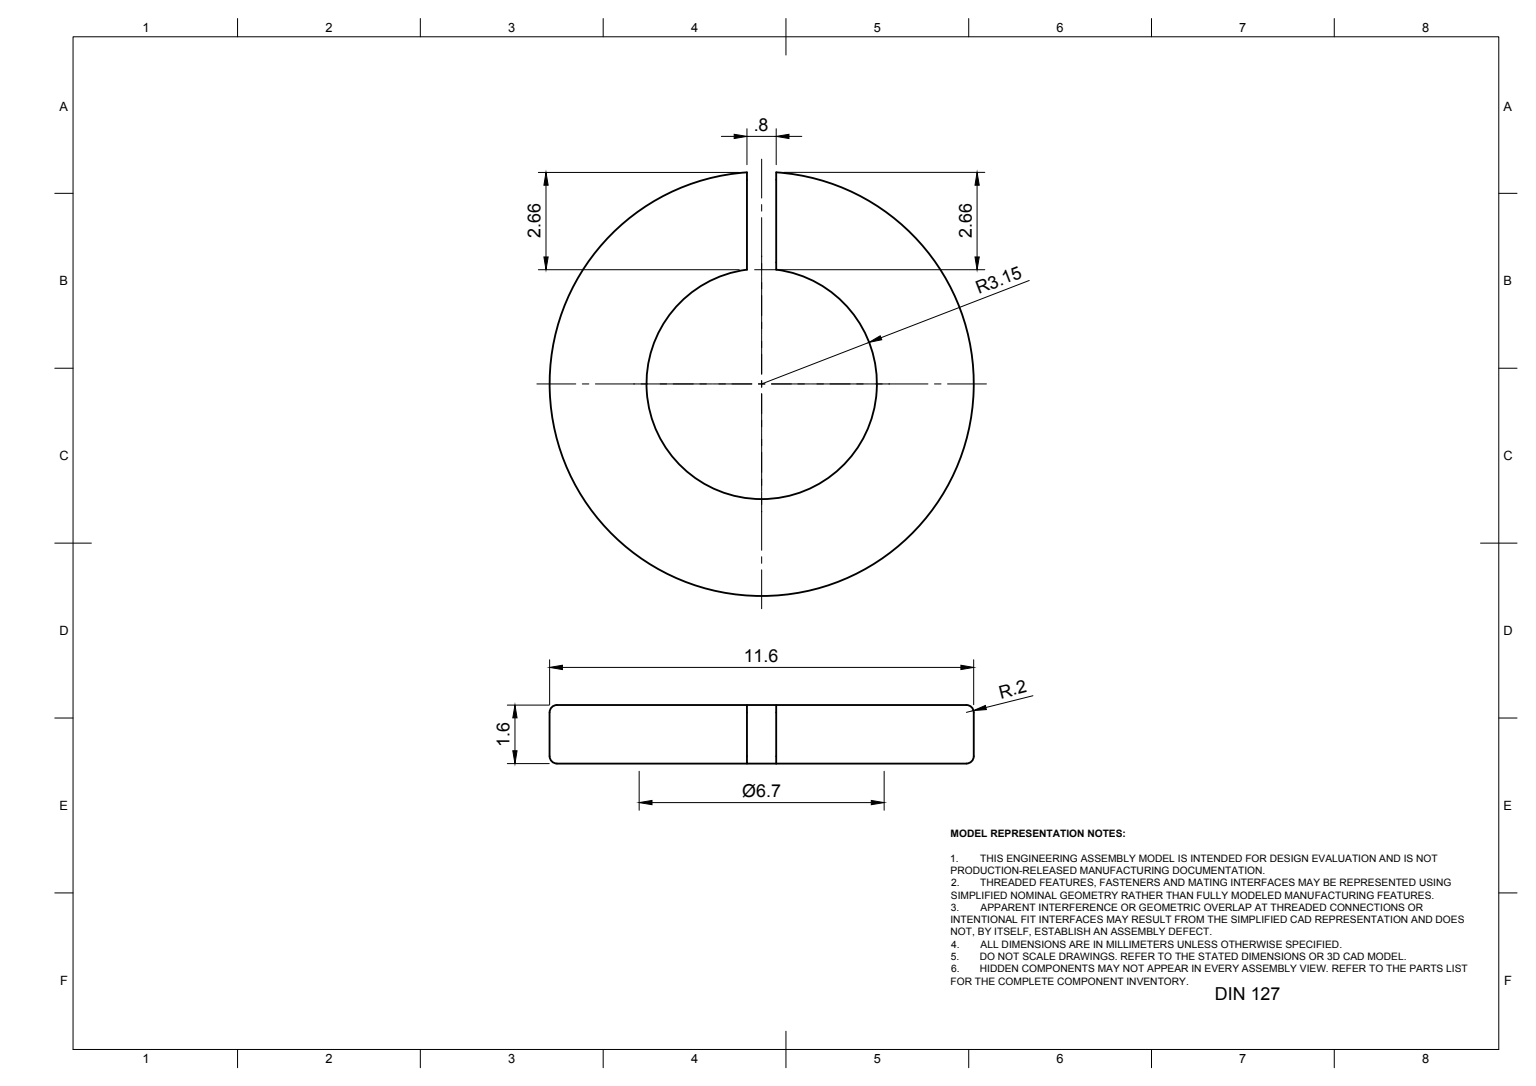
ISO-10303-21;
HEADER;
/* Generated by software containing ST-Developer
 * from STEP Tools, Inc. (www.steptools.com) 
 */

FILE_DESCRIPTION(
/* description */ ('STEP AP214'),
/* implementation_level */ '2;1');

FILE_NAME(
/* name */ 'DIN 127.step',
/* time_stamp */ '2026-10-07T12:18:07-07:00',
/* author */ (''),
/* organization */ (''),
/* preprocessor_version */ 'ST-DEVELOPER v20.2',
/* originating_system */ 'Autodesk Translation Framework v15.15.0.0',
/* authorisation */ '');

FILE_SCHEMA (('AUTOMOTIVE_DESIGN { 1 0 10303 214 3 1 1 }'));
ENDSEC;

DATA;
#10=MECHANICAL_DESIGN_GEOMETRIC_PRESENTATION_REPRESENTATION('',(#132),#62974);
#108=SHAPE_REPRESENTATION_RELATIONSHIP('SRR','None',#63031,#120);
#120=ADVANCED_BREP_SHAPE_REPRESENTATION('',(#144),#62972);
#132=STYLED_ITEM('',(#63090),#144);
#144=MANIFOLD_SOLID_BREP('Body1',#15202);
#716=PLANE('',#16878);
#717=PLANE('',#16879);
#718=PLANE('',#16882);
#719=PLANE('',#16883);
#1024=B_SPLINE_CURVE_WITH_KNOTS('',3,(#62662,#62663,#62664,#62665,#62666,
#62667,#62668,#62669,#62670,#62671),.UNSPECIFIED.,.F.,.F.,(4,2,2,2,4),(-0.0891808869303931,
-0.0817048501723883,-0.0742536419552704,-0.0668368032479844,-0.0594502997646748),
 .UNSPECIFIED.);
#1025=B_SPLINE_CURVE_WITH_KNOTS('',3,(#62674,#62675,#62676,#62677,#62678,
#62679,#62680,#62681,#62682,#62683),.UNSPECIFIED.,.F.,.F.,(4,2,2,2,4),(0.0594551317141721,
0.0668412192577732,0.0742583320696144,0.081710598423227,0.0891882604952256),
 .UNSPECIFIED.);
#1026=B_SPLINE_CURVE_WITH_KNOTS('',3,(#62689,#62690,#62691,#62692,#62693,
#62694,#62695,#62696,#62697,#62698),.UNSPECIFIED.,.F.,.F.,(4,2,2,2,4),(0.,
0.0073991168916538,0.0148071582868911,0.022226415171961,0.0296556575450588),
 .UNSPECIFIED.);
#1027=B_SPLINE_CURVE_WITH_KNOTS('',3,(#62701,#62702,#62703,#62704,#62705,
#62706,#62707,#62708,#62709,#62710),.UNSPECIFIED.,.F.,.F.,(4,2,2,2,4),(0.0889741245006404,
0.0964039199286515,0.103823503599454,0.111231617988348,0.118630606154988),
 .UNSPECIFIED.);
#1028=B_SPLINE_CURVE_WITH_KNOTS('',3,(#62716,#62717,#62718,#62719,#62720,
#62721,#62722,#62723,#62724,#62725),.UNSPECIFIED.,.F.,.F.,(4,2,2,2,4),(0.0889715481092505,
0.0964007904823484,0.103820047367418,0.111228088762656,0.118627205654309),
 .UNSPECIFIED.);
#1029=B_SPLINE_CURVE_WITH_KNOTS('',3,(#62728,#62729,#62730,#62731,#62732,
#62733,#62734,#62735,#62736,#62737),.UNSPECIFIED.,.F.,.F.,(4,2,2,2,4),(0.,
0.00739898816663991,0.014807102555534,0.0222266862263364,0.0296564816543475),
 .UNSPECIFIED.);
#1030=B_SPLINE_CURVE_WITH_KNOTS('',3,(#62743,#62744,#62745,#62746,#62747,
#62748,#62749,#62750,#62751,#62752),.UNSPECIFIED.,.F.,.F.,(4,2,2,2,4),(0.0594502997646748,
0.0668368032479844,0.0742536419552704,0.0817048501723883,0.0891808869303931),
 .UNSPECIFIED.);
#1031=B_SPLINE_CURVE_WITH_KNOTS('',3,(#62755,#62756,#62757,#62758,#62759,
#62760,#62761,#62762,#62763,#62764),.UNSPECIFIED.,.F.,.F.,(4,2,2,2,4),(0.0297220029331187,
0.0371996650051172,0.0446519313587299,0.0520690441705711,0.0594551317141721),
 .UNSPECIFIED.);
#2207=LINE('',#62766,#3400);
#2208=LINE('',#62767,#3401);
#2209=LINE('',#62769,#3402);
#2210=LINE('',#62770,#3403);
#2211=LINE('',#62772,#3404);
#2212=LINE('',#62773,#3405);
#2213=LINE('',#62775,#3406);
#2214=LINE('',#62776,#3407);
#3400=VECTOR('',#21190,1000.);
#3401=VECTOR('',#21191,1000.);
#3402=VECTOR('',#21194,1000.);
#3403=VECTOR('',#21195,1000.);
#3404=VECTOR('',#21198,1000.);
#3405=VECTOR('',#21199,1000.);
#3406=VECTOR('',#21202,1000.);
#3407=VECTOR('',#21203,1000.);
#3686=CYLINDRICAL_SURFACE('',#16880,3.15);
#3687=CYLINDRICAL_SURFACE('',#16881,5.8);
#4518=FACE_OUTER_BOUND('',#5468,.T.);
#4519=FACE_OUTER_BOUND('',#5469,.T.);
#4520=FACE_OUTER_BOUND('',#5470,.T.);
#4521=FACE_OUTER_BOUND('',#5471,.T.);
#4522=FACE_OUTER_BOUND('',#5472,.T.);
#4523=FACE_OUTER_BOUND('',#5473,.T.);
#4524=FACE_OUTER_BOUND('',#5474,.T.);
#4525=FACE_OUTER_BOUND('',#5475,.T.);
#4526=FACE_OUTER_BOUND('',#5476,.T.);
#4527=FACE_OUTER_BOUND('',#5477,.T.);
#5468=EDGE_LOOP('',(#14069,#14070,#14071,#14072));
#5469=EDGE_LOOP('',(#14073,#14074,#14075,#14076));
#5470=EDGE_LOOP('',(#14077,#14078,#14079,#14080));
#5471=EDGE_LOOP('',(#14081,#14082,#14083,#14084));
#5472=EDGE_LOOP('',(#14085,#14086,#14087,#14088));
#5473=EDGE_LOOP('',(#14089,#14090,#14091,#14092));
#5474=EDGE_LOOP('',(#14093,#14094,#14095,#14096));
#5475=EDGE_LOOP('',(#14097,#14098,#14099,#14100));
#5476=EDGE_LOOP('',(#14101,#14102,#14103,#14104,#14105,#14106,#14107,#14108));
#5477=EDGE_LOOP('',(#14109,#14110,#14111,#14112,#14113,#14114,#14115,#14116));
#6186=CIRCLE('',#16867,3.15);
#6187=CIRCLE('',#16868,3.35);
#6188=CIRCLE('',#16870,5.6);
#6189=CIRCLE('',#16871,5.8);
#6190=CIRCLE('',#16873,5.8);
#6191=CIRCLE('',#16874,5.6);
#6192=CIRCLE('',#16876,3.35);
#6193=CIRCLE('',#16877,3.15);
#7564=VERTEX_POINT('',#62658);
#7565=VERTEX_POINT('',#62659);
#7566=VERTEX_POINT('',#62661);
#7567=VERTEX_POINT('',#62672);
#7568=VERTEX_POINT('',#62685);
#7569=VERTEX_POINT('',#62686);
#7570=VERTEX_POINT('',#62688);
#7571=VERTEX_POINT('',#62699);
#7572=VERTEX_POINT('',#62712);
#7573=VERTEX_POINT('',#62713);
#7574=VERTEX_POINT('',#62715);
#7575=VERTEX_POINT('',#62726);
#7576=VERTEX_POINT('',#62739);
#7577=VERTEX_POINT('',#62740);
#7578=VERTEX_POINT('',#62742);
#7579=VERTEX_POINT('',#62753);
#9741=EDGE_CURVE('',#7564,#7565,#6186,.T.);
#9742=EDGE_CURVE('',#7566,#7564,#1024,.T.);
#9743=EDGE_CURVE('',#7567,#7566,#6187,.T.);
#9744=EDGE_CURVE('',#7565,#7567,#1025,.T.);
#9745=EDGE_CURVE('',#7568,#7569,#6188,.T.);
#9746=EDGE_CURVE('',#7570,#7568,#1026,.T.);
#9747=EDGE_CURVE('',#7571,#7570,#6189,.T.);
#9748=EDGE_CURVE('',#7569,#7571,#1027,.T.);
#9749=EDGE_CURVE('',#7572,#7573,#6190,.T.);
#9750=EDGE_CURVE('',#7574,#7572,#1028,.T.);
#9751=EDGE_CURVE('',#7575,#7574,#6191,.T.);
#9752=EDGE_CURVE('',#7573,#7575,#1029,.T.);
#9753=EDGE_CURVE('',#7576,#7577,#6192,.T.);
#9754=EDGE_CURVE('',#7578,#7576,#1030,.T.);
#9755=EDGE_CURVE('',#7579,#7578,#6193,.T.);
#9756=EDGE_CURVE('',#7577,#7579,#1031,.T.);
#9757=EDGE_CURVE('',#7567,#7569,#2207,.T.);
#9758=EDGE_CURVE('',#7568,#7566,#2208,.T.);
#9759=EDGE_CURVE('',#7577,#7575,#2209,.T.);
#9760=EDGE_CURVE('',#7574,#7576,#2210,.T.);
#9761=EDGE_CURVE('',#7578,#7564,#2211,.T.);
#9762=EDGE_CURVE('',#7579,#7565,#2212,.T.);
#9763=EDGE_CURVE('',#7572,#7570,#2213,.T.);
#9764=EDGE_CURVE('',#7573,#7571,#2214,.T.);
#14069=ORIENTED_EDGE('',*,*,#9741,.F.);
#14070=ORIENTED_EDGE('',*,*,#9742,.F.);
#14071=ORIENTED_EDGE('',*,*,#9743,.F.);
#14072=ORIENTED_EDGE('',*,*,#9744,.F.);
#14073=ORIENTED_EDGE('',*,*,#9745,.F.);
#14074=ORIENTED_EDGE('',*,*,#9746,.F.);
#14075=ORIENTED_EDGE('',*,*,#9747,.F.);
#14076=ORIENTED_EDGE('',*,*,#9748,.F.);
#14077=ORIENTED_EDGE('',*,*,#9749,.F.);
#14078=ORIENTED_EDGE('',*,*,#9750,.F.);
#14079=ORIENTED_EDGE('',*,*,#9751,.F.);
#14080=ORIENTED_EDGE('',*,*,#9752,.F.);
#14081=ORIENTED_EDGE('',*,*,#9753,.F.);
#14082=ORIENTED_EDGE('',*,*,#9754,.F.);
#14083=ORIENTED_EDGE('',*,*,#9755,.F.);
#14084=ORIENTED_EDGE('',*,*,#9756,.F.);
#14085=ORIENTED_EDGE('',*,*,#9757,.F.);
#14086=ORIENTED_EDGE('',*,*,#9743,.T.);
#14087=ORIENTED_EDGE('',*,*,#9758,.F.);
#14088=ORIENTED_EDGE('',*,*,#9745,.T.);
#14089=ORIENTED_EDGE('',*,*,#9759,.T.);
#14090=ORIENTED_EDGE('',*,*,#9751,.T.);
#14091=ORIENTED_EDGE('',*,*,#9760,.T.);
#14092=ORIENTED_EDGE('',*,*,#9753,.T.);
#14093=ORIENTED_EDGE('',*,*,#9761,.T.);
#14094=ORIENTED_EDGE('',*,*,#9741,.T.);
#14095=ORIENTED_EDGE('',*,*,#9762,.F.);
#14096=ORIENTED_EDGE('',*,*,#9755,.T.);
#14097=ORIENTED_EDGE('',*,*,#9763,.F.);
#14098=ORIENTED_EDGE('',*,*,#9749,.T.);
#14099=ORIENTED_EDGE('',*,*,#9764,.T.);
#14100=ORIENTED_EDGE('',*,*,#9747,.T.);
#14101=ORIENTED_EDGE('',*,*,#9758,.T.);
#14102=ORIENTED_EDGE('',*,*,#9742,.T.);
#14103=ORIENTED_EDGE('',*,*,#9761,.F.);
#14104=ORIENTED_EDGE('',*,*,#9754,.T.);
#14105=ORIENTED_EDGE('',*,*,#9760,.F.);
#14106=ORIENTED_EDGE('',*,*,#9750,.T.);
#14107=ORIENTED_EDGE('',*,*,#9763,.T.);
#14108=ORIENTED_EDGE('',*,*,#9746,.T.);
#14109=ORIENTED_EDGE('',*,*,#9762,.T.);
#14110=ORIENTED_EDGE('',*,*,#9744,.T.);
#14111=ORIENTED_EDGE('',*,*,#9757,.T.);
#14112=ORIENTED_EDGE('',*,*,#9748,.T.);
#14113=ORIENTED_EDGE('',*,*,#9764,.F.);
#14114=ORIENTED_EDGE('',*,*,#9752,.T.);
#14115=ORIENTED_EDGE('',*,*,#9759,.F.);
#14116=ORIENTED_EDGE('',*,*,#9756,.T.);
#14318=TOROIDAL_SURFACE('',#16866,3.35,0.2);
#14319=TOROIDAL_SURFACE('',#16869,5.6,0.2);
#14320=TOROIDAL_SURFACE('',#16872,5.6,0.2);
#14321=TOROIDAL_SURFACE('',#16875,3.35,0.2);
#15153=ADVANCED_FACE('',(#4518),#14318,.T.);
#15154=ADVANCED_FACE('',(#4519),#14319,.T.);
#15155=ADVANCED_FACE('',(#4520),#14320,.T.);
#15156=ADVANCED_FACE('',(#4521),#14321,.T.);
#15157=ADVANCED_FACE('',(#4522),#716,.F.);
#15158=ADVANCED_FACE('',(#4523),#717,.T.);
#15159=ADVANCED_FACE('',(#4524),#3686,.F.);
#15160=ADVANCED_FACE('',(#4525),#3687,.T.);
#15161=ADVANCED_FACE('',(#4526),#718,.F.);
#15162=ADVANCED_FACE('',(#4527),#719,.F.);
#15202=CLOSED_SHELL('',(#15153,#15154,#15155,#15156,#15157,#15158,#15159,
#15160,#15161,#15162));
#16865=AXIS2_PLACEMENT_3D('',#62656,#21162,#21163);
#16866=AXIS2_PLACEMENT_3D('',#62657,#21164,#21165);
#16867=AXIS2_PLACEMENT_3D('',#62660,#21166,#21167);
#16868=AXIS2_PLACEMENT_3D('',#62673,#21168,#21169);
#16869=AXIS2_PLACEMENT_3D('',#62684,#21170,#21171);
#16870=AXIS2_PLACEMENT_3D('',#62687,#21172,#21173);
#16871=AXIS2_PLACEMENT_3D('',#62700,#21174,#21175);
#16872=AXIS2_PLACEMENT_3D('',#62711,#21176,#21177);
#16873=AXIS2_PLACEMENT_3D('',#62714,#21178,#21179);
#16874=AXIS2_PLACEMENT_3D('',#62727,#21180,#21181);
#16875=AXIS2_PLACEMENT_3D('',#62738,#21182,#21183);
#16876=AXIS2_PLACEMENT_3D('',#62741,#21184,#21185);
#16877=AXIS2_PLACEMENT_3D('',#62754,#21186,#21187);
#16878=AXIS2_PLACEMENT_3D('',#62765,#21188,#21189);
#16879=AXIS2_PLACEMENT_3D('',#62768,#21192,#21193);
#16880=AXIS2_PLACEMENT_3D('',#62771,#21196,#21197);
#16881=AXIS2_PLACEMENT_3D('',#62774,#21200,#21201);
#16882=AXIS2_PLACEMENT_3D('',#62777,#21204,#21205);
#16883=AXIS2_PLACEMENT_3D('',#62778,#21206,#21207);
#21162=DIRECTION('axis',(0.,0.,1.));
#21163=DIRECTION('refdir',(1.,0.,0.));
#21164=DIRECTION('center_axis',(0.,-1.,0.));
#21165=DIRECTION('ref_axis',(-1.,0.,0.));
#21166=DIRECTION('center_axis',(0.,1.,0.));
#21167=DIRECTION('ref_axis',(-1.,0.,0.));
#21168=DIRECTION('center_axis',(0.,-1.,0.));
#21169=DIRECTION('ref_axis',(-1.,0.,0.));
#21170=DIRECTION('center_axis',(0.,-1.,0.));
#21171=DIRECTION('ref_axis',(-1.,0.,0.));
#21172=DIRECTION('center_axis',(0.,1.,0.));
#21173=DIRECTION('ref_axis',(-1.,0.,0.));
#21174=DIRECTION('center_axis',(0.,-1.,0.));
#21175=DIRECTION('ref_axis',(-1.,0.,0.));
#21176=DIRECTION('center_axis',(0.,-1.,0.));
#21177=DIRECTION('ref_axis',(-1.,0.,0.));
#21178=DIRECTION('center_axis',(0.,1.,0.));
#21179=DIRECTION('ref_axis',(-1.,0.,0.));
#21180=DIRECTION('center_axis',(0.,-1.,0.));
#21181=DIRECTION('ref_axis',(-1.,0.,0.));
#21182=DIRECTION('center_axis',(0.,-1.,0.));
#21183=DIRECTION('ref_axis',(-1.,0.,0.));
#21184=DIRECTION('center_axis',(0.,1.,0.));
#21185=DIRECTION('ref_axis',(-1.,0.,0.));
#21186=DIRECTION('center_axis',(0.,-1.,0.));
#21187=DIRECTION('ref_axis',(-1.,0.,0.));
#21188=DIRECTION('center_axis',(0.,-1.,0.));
#21189=DIRECTION('ref_axis',(0.,0.,1.));
#21190=DIRECTION('',(1.,0.,0.));
#21191=DIRECTION('',(-1.,0.,1.32390688747943E-15));
#21192=DIRECTION('center_axis',(0.,-1.,0.));
#21193=DIRECTION('ref_axis',(0.,0.,1.));
#21194=DIRECTION('',(1.,0.,0.));
#21195=DIRECTION('',(-1.,0.,1.32390688747943E-15));
#21196=DIRECTION('center_axis',(0.,-1.,0.));
#21197=DIRECTION('ref_axis',(-0.999999745434011,0.,-0.000713534802215152));
#21198=DIRECTION('',(0.,1.,0.));
#21199=DIRECTION('',(0.,1.,0.));
#21200=DIRECTION('center_axis',(0.,-1.,0.));
#21201=DIRECTION('ref_axis',(-0.999999925770602,0.,-0.000385303503088288));
#21202=DIRECTION('',(0.,1.,0.));
#21203=DIRECTION('',(0.,1.,0.));
#21204=DIRECTION('center_axis',(-1.32390688747943E-15,0.,-1.));
#21205=DIRECTION('ref_axis',(1.,0.,-1.32390688747943E-15));
#21206=DIRECTION('center_axis',(0.,0.,1.));
#21207=DIRECTION('ref_axis',(0.,-1.,0.));
#62656=CARTESIAN_POINT('',(0.,0.,0.));
#62657=CARTESIAN_POINT('Origin',(0.,51.8,23.999999203644));
#62658=CARTESIAN_POINT('',(3.12478456555985,51.8,23.6022286430957));
#62659=CARTESIAN_POINT('',(3.12421373757276,51.8,24.4022286430957));
#62660=CARTESIAN_POINT('Origin',(0.,51.8,23.999999203644));
#62661=CARTESIAN_POINT('',(3.32630103585967,52.,23.6022286430957));
#62662=CARTESIAN_POINT('Ctrl Pts',(3.32630103585966,52.,23.6022286430957));
#62663=CARTESIAN_POINT('Ctrl Pts',(3.30138091333298,52.,23.6022286430957));
#62664=CARTESIAN_POINT('Ctrl Pts',(3.2720456700574,51.9941946996912,23.6022286430957));
#62665=CARTESIAN_POINT('Ctrl Pts',(3.22604606522074,51.9752251584662,23.6022286430957));
#62666=CARTESIAN_POINT('Ctrl Pts',(3.20122053120427,51.9587321016509,23.6022286430957));
#62667=CARTESIAN_POINT('Ctrl Pts',(3.1660925751105,51.9237716124592,23.6022286430957));
#62668=CARTESIAN_POINT('Ctrl Pts',(3.14954178912886,51.8991500075979,23.6022286430957));
#62669=CARTESIAN_POINT('Ctrl Pts',(3.13058236701996,51.853593258103,23.6022286430957));
#62670=CARTESIAN_POINT('Ctrl Pts',(3.12478456555985,51.8246216782777,23.6022286430957));
#62671=CARTESIAN_POINT('Ctrl Pts',(3.12478456555985,51.8,23.6022286430957));
#62672=CARTESIAN_POINT('',(3.32576479595873,52.,24.4022286430957));
#62673=CARTESIAN_POINT('Origin',(0.,52.,23.999999203644));
#62674=CARTESIAN_POINT('Ctrl Pts',(3.12421373757277,51.8,24.4022286430957));
#62675=CARTESIAN_POINT('Ctrl Pts',(3.12421373757277,51.824620291812,24.4022286430957));
#62676=CARTESIAN_POINT('Ctrl Pts',(3.13001197949707,51.8535900867339,24.4022286430957));
#62677=CARTESIAN_POINT('Ctrl Pts',(3.1489729516324,51.8991456790208,24.4022286430957));
#62678=CARTESIAN_POINT('Ctrl Pts',(3.16552590642155,51.9237671470348,24.4022286430957));
#62679=CARTESIAN_POINT('Ctrl Pts',(3.20065890912318,51.9587288606451,24.4022286430957));
#62680=CARTESIAN_POINT('Ctrl Pts',(3.2254889592639,51.9752227683353,24.4022286430957));
#62681=CARTESIAN_POINT('Ctrl Pts',(3.27149750609936,51.9941940883332,24.4022286430957));
#62682=CARTESIAN_POINT('Ctrl Pts',(3.30083925571873,52.,24.4022286430957));
#62683=CARTESIAN_POINT('Ctrl Pts',(3.32576479595873,52.,24.4022286430957));
#62684=CARTESIAN_POINT('Origin',(3.30681662608079E-15,51.8,23.999999203644));
#62685=CARTESIAN_POINT('',(5.58585522379171,52.,23.6022286430957));
#62686=CARTESIAN_POINT('',(5.58553591681572,52.,24.4022286430957));
#62687=CARTESIAN_POINT('Origin',(3.30681662608079E-15,52.,23.999999203644));
#62688=CARTESIAN_POINT('',(5.78634414645043,51.8,23.6022286430957));
#62689=CARTESIAN_POINT('Ctrl Pts',(5.78634414645042,51.8,23.6022286430957));
#62690=CARTESIAN_POINT('Ctrl Pts',(5.78634414645042,51.8246637229722,23.6022286430957));
#62691=CARTESIAN_POINT('Ctrl Pts',(5.78056058173252,51.8536895954238,23.6022286430957));
#62692=CARTESIAN_POINT('Ctrl Pts',(5.76165032214247,51.8992805452974,23.6022286430957));
#62693=CARTESIAN_POINT('Ctrl Pts',(5.74516733469338,51.923905255687,23.6022286430957));
#62694=CARTESIAN_POINT('Ctrl Pts',(5.71019378482186,51.958828241931,23.6022286430957));
#62695=CARTESIAN_POINT('Ctrl Pts',(5.68550434648015,51.9752951055667,23.6022286430957));
#62696=CARTESIAN_POINT('Ctrl Pts',(5.63976742956776,51.9942130655933,23.6022286430957));
#62697=CARTESIAN_POINT('Ctrl Pts',(5.61061936503537,52.,23.6022286430957));
#62698=CARTESIAN_POINT('Ctrl Pts',(5.58585522379171,52.,23.6022286430957));
#62699=CARTESIAN_POINT('',(5.78603590362507,51.8,24.4022286430957));
#62700=CARTESIAN_POINT('Origin',(3.30681662608079E-15,51.8,23.999999203644));
#62701=CARTESIAN_POINT('Ctrl Pts',(5.58553591681572,52.,24.4022286430957));
#62702=CARTESIAN_POINT('Ctrl Pts',(5.61030190157576,52.,24.4022286430957));
#62703=CARTESIAN_POINT('Ctrl Pts',(5.63945218333164,51.9942128733221,24.4022286430957));
#62704=CARTESIAN_POINT('Ctrl Pts',(5.68519202491141,51.9752943110313,24.4022286430957));
#62705=CARTESIAN_POINT('Ctrl Pts',(5.70988286438085,51.9588271924047,24.4022286430957));
#62706=CARTESIAN_POINT('Ctrl Pts',(5.7448579281656,51.9239038363323,24.4022286430957));
#62707=CARTESIAN_POINT('Ctrl Pts',(5.76134153541181,51.8992791894732,24.4022286430957));
#62708=CARTESIAN_POINT('Ctrl Pts',(5.78025222289073,51.8536886182006,24.4022286430957));
#62709=CARTESIAN_POINT('Ctrl Pts',(5.78603590362507,51.8246632938888,24.4022286430957));
#62710=CARTESIAN_POINT('Ctrl Pts',(5.78603590362507,51.8,24.4022286430957));
#62711=CARTESIAN_POINT('Origin',(3.30681662608079E-15,50.6,23.999999203644));
#62712=CARTESIAN_POINT('',(5.78634414645043,50.6,23.6022286430957));
#62713=CARTESIAN_POINT('',(5.78603590362507,50.6,24.4022286430957));
#62714=CARTESIAN_POINT('Origin',(3.30681662608079E-15,50.6,23.999999203644));
#62715=CARTESIAN_POINT('',(5.58585522379171,50.4,23.6022286430957));
#62716=CARTESIAN_POINT('Ctrl Pts',(5.5858552237917,50.4,23.6022286430957));
#62717=CARTESIAN_POINT('Ctrl Pts',(5.61061936503536,50.4,23.6022286430957));
#62718=CARTESIAN_POINT('Ctrl Pts',(5.63976742956776,50.4057869344067,23.6022286430957));
#62719=CARTESIAN_POINT('Ctrl Pts',(5.68550434648015,50.4247048944333,23.6022286430957));
#62720=CARTESIAN_POINT('Ctrl Pts',(5.71019378482186,50.441171758069,23.6022286430957));
#62721=CARTESIAN_POINT('Ctrl Pts',(5.74516733469338,50.476094744313,23.6022286430957));
#62722=CARTESIAN_POINT('Ctrl Pts',(5.76165032214247,50.5007194547026,23.6022286430957));
#62723=CARTESIAN_POINT('Ctrl Pts',(5.78056058173252,50.5463104045762,23.6022286430957));
#62724=CARTESIAN_POINT('Ctrl Pts',(5.78634414645042,50.5753362770278,23.6022286430957));
#62725=CARTESIAN_POINT('Ctrl Pts',(5.78634414645042,50.6,23.6022286430957));
#62726=CARTESIAN_POINT('',(5.58553591681572,50.4,24.4022286430957));
#62727=CARTESIAN_POINT('Origin',(3.30681662608079E-15,50.4,23.999999203644));
#62728=CARTESIAN_POINT('Ctrl Pts',(5.78603590362507,50.6,24.4022286430957));
#62729=CARTESIAN_POINT('Ctrl Pts',(5.78603590362507,50.5753367061112,24.4022286430957));
#62730=CARTESIAN_POINT('Ctrl Pts',(5.78025222289073,50.5463113817994,24.4022286430957));
#62731=CARTESIAN_POINT('Ctrl Pts',(5.76134153541181,50.5007208105268,24.4022286430957));
#62732=CARTESIAN_POINT('Ctrl Pts',(5.7448579281656,50.4760961636677,24.4022286430957));
#62733=CARTESIAN_POINT('Ctrl Pts',(5.70988286438085,50.4411728075953,24.4022286430957));
#62734=CARTESIAN_POINT('Ctrl Pts',(5.68519202491141,50.4247056889687,24.4022286430957));
#62735=CARTESIAN_POINT('Ctrl Pts',(5.63945218333164,50.4057871266779,24.4022286430957));
#62736=CARTESIAN_POINT('Ctrl Pts',(5.61030190157576,50.4,24.4022286430957));
#62737=CARTESIAN_POINT('Ctrl Pts',(5.58553591681572,50.4,24.4022286430957));
#62738=CARTESIAN_POINT('Origin',(0.,50.6,23.999999203644));
#62739=CARTESIAN_POINT('',(3.32630103585967,50.4,23.6022286430957));
#62740=CARTESIAN_POINT('',(3.32576479595873,50.4,24.4022286430957));
#62741=CARTESIAN_POINT('Origin',(0.,50.4,23.999999203644));
#62742=CARTESIAN_POINT('',(3.12478456555985,50.6,23.6022286430957));
#62743=CARTESIAN_POINT('Ctrl Pts',(3.12478456555985,50.6,23.6022286430957));
#62744=CARTESIAN_POINT('Ctrl Pts',(3.12478456555985,50.5753783217223,23.6022286430957));
#62745=CARTESIAN_POINT('Ctrl Pts',(3.13058236701996,50.546406741897,23.6022286430957));
#62746=CARTESIAN_POINT('Ctrl Pts',(3.14954178912886,50.5008499924022,23.6022286430957));
#62747=CARTESIAN_POINT('Ctrl Pts',(3.1660925751105,50.4762283875408,23.6022286430957));
#62748=CARTESIAN_POINT('Ctrl Pts',(3.20122053120427,50.4412678983491,23.6022286430957));
#62749=CARTESIAN_POINT('Ctrl Pts',(3.22604606522074,50.4247748415338,23.6022286430957));
#62750=CARTESIAN_POINT('Ctrl Pts',(3.2720456700574,50.4058053003088,23.6022286430957));
#62751=CARTESIAN_POINT('Ctrl Pts',(3.30138091333298,50.4,23.6022286430957));
#62752=CARTESIAN_POINT('Ctrl Pts',(3.32630103585966,50.4,23.6022286430957));
#62753=CARTESIAN_POINT('',(3.12421373757276,50.6,24.4022286430957));
#62754=CARTESIAN_POINT('Origin',(0.,50.6,23.999999203644));
#62755=CARTESIAN_POINT('Ctrl Pts',(3.32576479595873,50.4,24.4022286430957));
#62756=CARTESIAN_POINT('Ctrl Pts',(3.30083925571873,50.4,24.4022286430957));
#62757=CARTESIAN_POINT('Ctrl Pts',(3.27149750609936,50.4058059116668,24.4022286430957));
#62758=CARTESIAN_POINT('Ctrl Pts',(3.2254889592639,50.4247772316647,24.4022286430957));
#62759=CARTESIAN_POINT('Ctrl Pts',(3.20065890912318,50.4412711393549,24.4022286430957));
#62760=CARTESIAN_POINT('Ctrl Pts',(3.16552590642155,50.4762328529652,24.4022286430957));
#62761=CARTESIAN_POINT('Ctrl Pts',(3.1489729516324,50.5008543209792,24.4022286430957));
#62762=CARTESIAN_POINT('Ctrl Pts',(3.13001197949707,50.5464099132661,24.4022286430957));
#62763=CARTESIAN_POINT('Ctrl Pts',(3.12421373757277,50.575379708188,24.4022286430957));
#62764=CARTESIAN_POINT('Ctrl Pts',(3.12421373757277,50.6,24.4022286430957));
#62765=CARTESIAN_POINT('Origin',(3.30681662608079E-15,52.,23.999999203644));
#62766=CARTESIAN_POINT('',(5.78603590362507,52.,24.4022286430957));
#62767=CARTESIAN_POINT('',(3.12478456555985,52.,23.6022286430957));
#62768=CARTESIAN_POINT('Origin',(3.30681662608079E-15,50.4,23.999999203644));
#62769=CARTESIAN_POINT('',(5.78603590362507,50.4,24.4022286430957));
#62770=CARTESIAN_POINT('',(3.12478456555985,50.4,23.6022286430957));
#62771=CARTESIAN_POINT('Origin',(0.,50.4,23.999999203644));
#62772=CARTESIAN_POINT('',(3.12478456555985,50.4,23.6022286430957));
#62773=CARTESIAN_POINT('',(3.12421373757276,50.4,24.4022286430957));
#62774=CARTESIAN_POINT('Origin',(3.30681662608079E-15,50.4,23.999999203644));
#62775=CARTESIAN_POINT('',(5.78634414645043,50.4,23.6022286430957));
#62776=CARTESIAN_POINT('',(5.78603590362507,50.4,24.4022286430957));
#62777=CARTESIAN_POINT('Origin',(3.12478456555985,50.4,23.6022286430957));
#62778=CARTESIAN_POINT('Origin',(5.78603590362507,50.4,24.4022286430957));
#62958=UNCERTAINTY_MEASURE_WITH_UNIT(LENGTH_MEASURE(0.01),#62975,
'DISTANCE_ACCURACY_VALUE',
'Maximum model space distance between geometric entities at asserted c
onnectivities');
#62960=UNCERTAINTY_MEASURE_WITH_UNIT(LENGTH_MEASURE(0.01),#62975,
'DISTANCE_ACCURACY_VALUE',
'Maximum model space distance between geometric entities at asserted c
onnectivities');
#62972=(
GEOMETRIC_REPRESENTATION_CONTEXT(3)
GLOBAL_UNCERTAINTY_ASSIGNED_CONTEXT((#62958))
GLOBAL_UNIT_ASSIGNED_CONTEXT((#62975,#62977,#62978))
REPRESENTATION_CONTEXT('','3D')
);
#62974=(
GEOMETRIC_REPRESENTATION_CONTEXT(3)
GLOBAL_UNCERTAINTY_ASSIGNED_CONTEXT((#62960))
GLOBAL_UNIT_ASSIGNED_CONTEXT((#62975,#62977,#62978))
REPRESENTATION_CONTEXT('','3D')
);
#62975=(
LENGTH_UNIT()
NAMED_UNIT(*)
SI_UNIT(.MILLI.,.METRE.)
);
#62977=(
NAMED_UNIT(*)
PLANE_ANGLE_UNIT()
SI_UNIT($,.RADIAN.)
);
#62978=(
NAMED_UNIT(*)
SI_UNIT($,.STERADIAN.)
SOLID_ANGLE_UNIT()
);
#62990=SHAPE_DEFINITION_REPRESENTATION(#63003,#63031);
#63003=PRODUCT_DEFINITION_SHAPE('',$,#63045);
#63031=SHAPE_REPRESENTATION('',(#16865),#62972);
#63033=PRODUCT_DEFINITION_CONTEXT('part definition',#63074,'design');
#63045=PRODUCT_DEFINITION('DIN 127','DIN 127',#63058,#63033);
#63058=PRODUCT_DEFINITION_FORMATION('',$,#63087);
#63074=APPLICATION_CONTEXT(
'Core Data for Automotive Mechanical Design Process');
#63075=PRODUCT_CONTEXT('part definition',#63074,'mechanical');
#63087=PRODUCT('DIN 127','DIN 127',$,(#63075));
#63090=PRESENTATION_STYLE_ASSIGNMENT((#63092));
#63092=SURFACE_STYLE_USAGE(.BOTH.,#63094);
#63094=SURFACE_SIDE_STYLE('',(#63096));
#63096=SURFACE_STYLE_FILL_AREA(#63098);
#63098=FILL_AREA_STYLE('Opaque(202,209,238)',(#63100));
#63100=FILL_AREA_STYLE_COLOUR('Opaque(202,209,238)',#63102);
#63102=COLOUR_RGB('Opaque(202,209,238)', 0.66274510, 0.83137255, 0.94901961);
ENDSEC;
END-ISO-10303-21;
